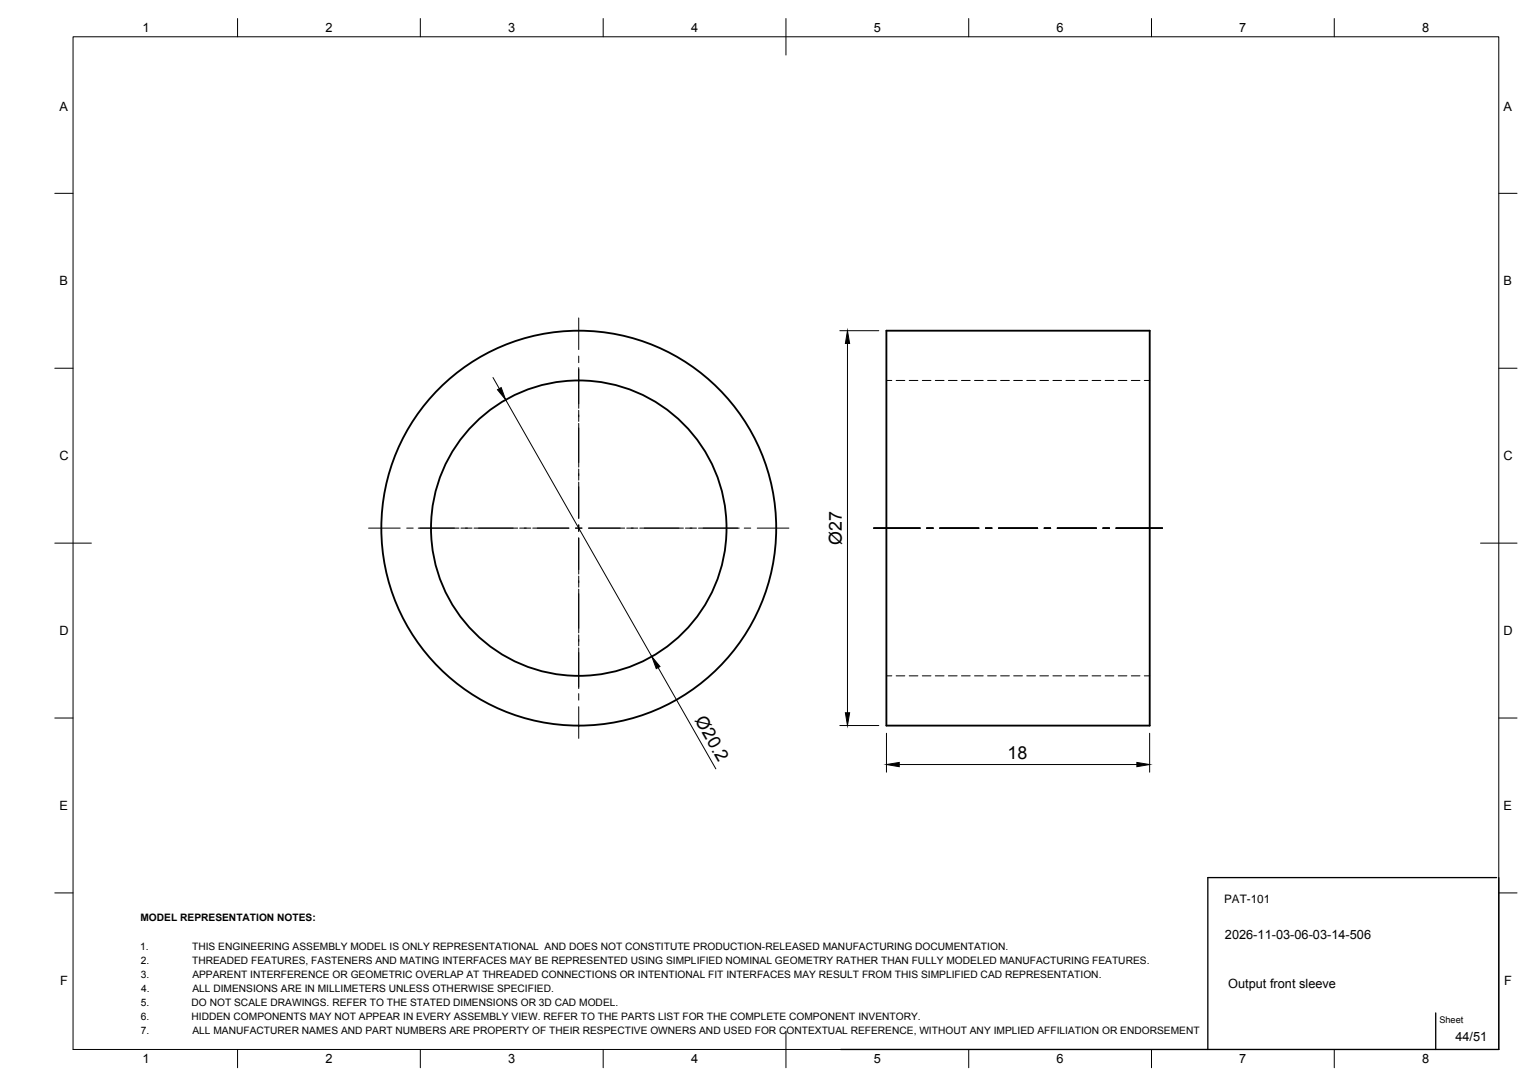
ISO-10303-21;
HEADER;
/* Generated by software containing ST-Developer
 * from STEP Tools, Inc. (www.steptools.com) 
 */

FILE_DESCRIPTION(
/* description */ ('Spur gear reduction stage 2-1 on bearing plates'),
/* implementation_level */ '2;1');

FILE_NAME(
/* name */ 'Output front sleeve.step',
/* time_stamp */ '2026-10-28T03:22:07-07:00',
/* author */ (''),
/* organization */ (''),
/* preprocessor_version */ 'ST-DEVELOPER v20.2',
/* originating_system */ 'Autodesk Translation Framework v15.17.0.0',
/* authorisation */ '');

FILE_SCHEMA (('AUTOMOTIVE_DESIGN { 1 0 10303 214 3 1 1 }'));
ENDSEC;

DATA;
#10=MECHANICAL_DESIGN_GEOMETRIC_PRESENTATION_REPRESENTATION('',(#996),#53909);
#895=SHAPE_REPRESENTATION_RELATIONSHIP('SRR','None',#54126,#938);
#938=ADVANCED_BREP_SHAPE_REPRESENTATION('',(#1051),#53900);
#996=STYLED_ITEM('',(#54411),#1051);
#1051=MANIFOLD_SOLID_BREP('Body1',#11323);
#1218=FACE_BOUND('',#2740,.T.);
#1219=FACE_BOUND('',#2742,.T.);
#1422=PLANE('',#12697);
#1423=PLANE('',#12698);
#1931=FACE_OUTER_BOUND('',#2737,.T.);
#1932=FACE_OUTER_BOUND('',#2738,.T.);
#1933=FACE_OUTER_BOUND('',#2739,.T.);
#1934=FACE_OUTER_BOUND('',#2741,.T.);
#2737=EDGE_LOOP('',(#9220,#9221,#9222,#9223));
#2738=EDGE_LOOP('',(#9224,#9225,#9226,#9227));
#2739=EDGE_LOOP('',(#9228));
#2740=EDGE_LOOP('',(#9229));
#2741=EDGE_LOOP('',(#9230));
#2742=EDGE_LOOP('',(#9231));
#3384=LINE('',#29881,#4025);
#3385=LINE('',#29887,#4026);
#4025=VECTOR('',#15163,1.01);
#4026=VECTOR('',#15170,1.35);
#4666=CIRCLE('',#12692,1.01);
#4667=CIRCLE('',#12693,1.01);
#4668=CIRCLE('',#12695,1.35);
#4669=CIRCLE('',#12696,1.35);
#5418=VERTEX_POINT('',#29878);
#5419=VERTEX_POINT('',#29880);
#5420=VERTEX_POINT('',#29884);
#5421=VERTEX_POINT('',#29886);
#6752=EDGE_CURVE('',#5418,#5418,#4666,.T.);
#6753=EDGE_CURVE('',#5418,#5419,#3384,.T.);
#6754=EDGE_CURVE('',#5419,#5419,#4667,.T.);
#6755=EDGE_CURVE('',#5420,#5420,#4668,.T.);
#6756=EDGE_CURVE('',#5420,#5421,#3385,.T.);
#6757=EDGE_CURVE('',#5421,#5421,#4669,.T.);
#9220=ORIENTED_EDGE('',*,*,#6752,.F.);
#9221=ORIENTED_EDGE('',*,*,#6753,.T.);
#9222=ORIENTED_EDGE('',*,*,#6754,.T.);
#9223=ORIENTED_EDGE('',*,*,#6753,.F.);
#9224=ORIENTED_EDGE('',*,*,#6755,.F.);
#9225=ORIENTED_EDGE('',*,*,#6756,.T.);
#9226=ORIENTED_EDGE('',*,*,#6757,.T.);
#9227=ORIENTED_EDGE('',*,*,#6756,.F.);
#9228=ORIENTED_EDGE('',*,*,#6755,.T.);
#9229=ORIENTED_EDGE('',*,*,#6752,.T.);
#9230=ORIENTED_EDGE('',*,*,#6757,.F.);
#9231=ORIENTED_EDGE('',*,*,#6754,.F.);
#10566=CYLINDRICAL_SURFACE('',#12691,1.01);
#10567=CYLINDRICAL_SURFACE('',#12694,1.35);
#11051=ADVANCED_FACE('',(#1931),#10566,.F.);
#11052=ADVANCED_FACE('',(#1932),#10567,.T.);
#11053=ADVANCED_FACE('',(#1933,#1218),#1422,.T.);
#11054=ADVANCED_FACE('',(#1934,#1219),#1423,.F.);
#11323=CLOSED_SHELL('',(#11051,#11052,#11053,#11054));
#12690=AXIS2_PLACEMENT_3D('',#29876,#15157,#15158);
#12691=AXIS2_PLACEMENT_3D('',#29877,#15159,#15160);
#12692=AXIS2_PLACEMENT_3D('',#29879,#15161,#15162);
#12693=AXIS2_PLACEMENT_3D('',#29882,#15164,#15165);
#12694=AXIS2_PLACEMENT_3D('',#29883,#15166,#15167);
#12695=AXIS2_PLACEMENT_3D('',#29885,#15168,#15169);
#12696=AXIS2_PLACEMENT_3D('',#29888,#15171,#15172);
#12697=AXIS2_PLACEMENT_3D('',#29889,#15173,#15174);
#12698=AXIS2_PLACEMENT_3D('',#29890,#15175,#15176);
#15157=DIRECTION('axis',(0.,0.,1.));
#15158=DIRECTION('refdir',(1.,0.,0.));
#15159=DIRECTION('center_axis',(0.,1.,0.));
#15160=DIRECTION('ref_axis',(1.,0.,0.));
#15161=DIRECTION('center_axis',(0.,-1.,0.));
#15162=DIRECTION('ref_axis',(1.,0.,0.));
#15163=DIRECTION('',(0.,-1.,0.));
#15164=DIRECTION('center_axis',(0.,-1.,0.));
#15165=DIRECTION('ref_axis',(1.,0.,0.));
#15166=DIRECTION('center_axis',(0.,1.,0.));
#15167=DIRECTION('ref_axis',(1.,0.,0.));
#15168=DIRECTION('center_axis',(0.,1.,0.));
#15169=DIRECTION('ref_axis',(1.,0.,0.));
#15170=DIRECTION('',(0.,-1.,0.));
#15171=DIRECTION('center_axis',(0.,1.,0.));
#15172=DIRECTION('ref_axis',(1.,0.,0.));
#15173=DIRECTION('center_axis',(0.,1.,0.));
#15174=DIRECTION('ref_axis',(1.,0.,0.));
#15175=DIRECTION('center_axis',(0.,1.,0.));
#15176=DIRECTION('ref_axis',(1.,0.,0.));
#29876=CARTESIAN_POINT('',(0.,0.,0.));
#29877=CARTESIAN_POINT('Origin',(0.,-2.8,0.));
#29878=CARTESIAN_POINT('',(-1.01,-1.,1.23689326713883E-16));
#29879=CARTESIAN_POINT('Origin',(0.,-1.,0.));
#29880=CARTESIAN_POINT('',(-1.01,-2.8,1.23689326713883E-16));
#29881=CARTESIAN_POINT('',(-1.01,-2.8,1.23689326713883E-16));
#29882=CARTESIAN_POINT('Origin',(0.,-2.8,0.));
#29883=CARTESIAN_POINT('Origin',(0.,-2.8,0.));
#29884=CARTESIAN_POINT('',(-1.35,-1.,1.65327317884893E-16));
#29885=CARTESIAN_POINT('Origin',(0.,-1.,0.));
#29886=CARTESIAN_POINT('',(-1.35,-2.8,1.65327317884893E-16));
#29887=CARTESIAN_POINT('',(-1.35,-2.8,1.65327317884893E-16));
#29888=CARTESIAN_POINT('Origin',(0.,-2.8,0.));
#29889=CARTESIAN_POINT('Origin',(0.,-1.,0.));
#29890=CARTESIAN_POINT('Origin',(0.,-2.8,0.));
#53850=UNCERTAINTY_MEASURE_WITH_UNIT(LENGTH_MEASURE(0.001),#53910,
'DISTANCE_ACCURACY_VALUE',
'Maximum model space distance between geometric entities at asserted c
onnectivities');
#53859=UNCERTAINTY_MEASURE_WITH_UNIT(LENGTH_MEASURE(0.001),#53910,
'DISTANCE_ACCURACY_VALUE',
'Maximum model space distance between geometric entities at asserted c
onnectivities');
#53900=(
GEOMETRIC_REPRESENTATION_CONTEXT(3)
GLOBAL_UNCERTAINTY_ASSIGNED_CONTEXT((#53850))
GLOBAL_UNIT_ASSIGNED_CONTEXT((#53910,#53912,#53913))
REPRESENTATION_CONTEXT('','3D')
);
#53909=(
GEOMETRIC_REPRESENTATION_CONTEXT(3)
GLOBAL_UNCERTAINTY_ASSIGNED_CONTEXT((#53859))
GLOBAL_UNIT_ASSIGNED_CONTEXT((#53910,#53912,#53913))
REPRESENTATION_CONTEXT('','3D')
);
#53910=(
LENGTH_UNIT()
NAMED_UNIT(*)
SI_UNIT(.CENTI.,.METRE.)
);
#53912=(
NAMED_UNIT(*)
PLANE_ANGLE_UNIT()
SI_UNIT($,.RADIAN.)
);
#53913=(
NAMED_UNIT(*)
SI_UNIT($,.STERADIAN.)
SOLID_ANGLE_UNIT()
);
#53954=SHAPE_DEFINITION_REPRESENTATION(#54052,#54126);
#54052=PRODUCT_DEFINITION_SHAPE('',$,#54176);
#54126=SHAPE_REPRESENTATION('',(#12690),#53900);
#54135=PRODUCT_DEFINITION_CONTEXT('part definition',#54284,'design');
#54176=PRODUCT_DEFINITION('Output front sleeve','Output front sleeve',#54225,
#54135);
#54225=PRODUCT_DEFINITION_FORMATION('',$,#54326);
#54284=APPLICATION_CONTEXT(
'Core Data for Automotive Mechanical Design Process');
#54285=PRODUCT_CONTEXT('part definition',#54284,'mechanical');
#54326=PRODUCT('Output front sleeve','Output front sleeve',
'Output front sleeve',(#54285));
#54405=COLOUR_RGB('Off White',0.89,0.88,0.83);
#54406=FILL_AREA_STYLE_COLOUR('',#54405);
#54407=FILL_AREA_STYLE('',(#54406));
#54408=SURFACE_STYLE_FILL_AREA(#54407);
#54409=SURFACE_SIDE_STYLE('',(#54408));
#54410=SURFACE_STYLE_USAGE(.BOTH.,#54409);
#54411=PRESENTATION_STYLE_ASSIGNMENT((#54410));
ENDSEC;
END-ISO-10303-21;
